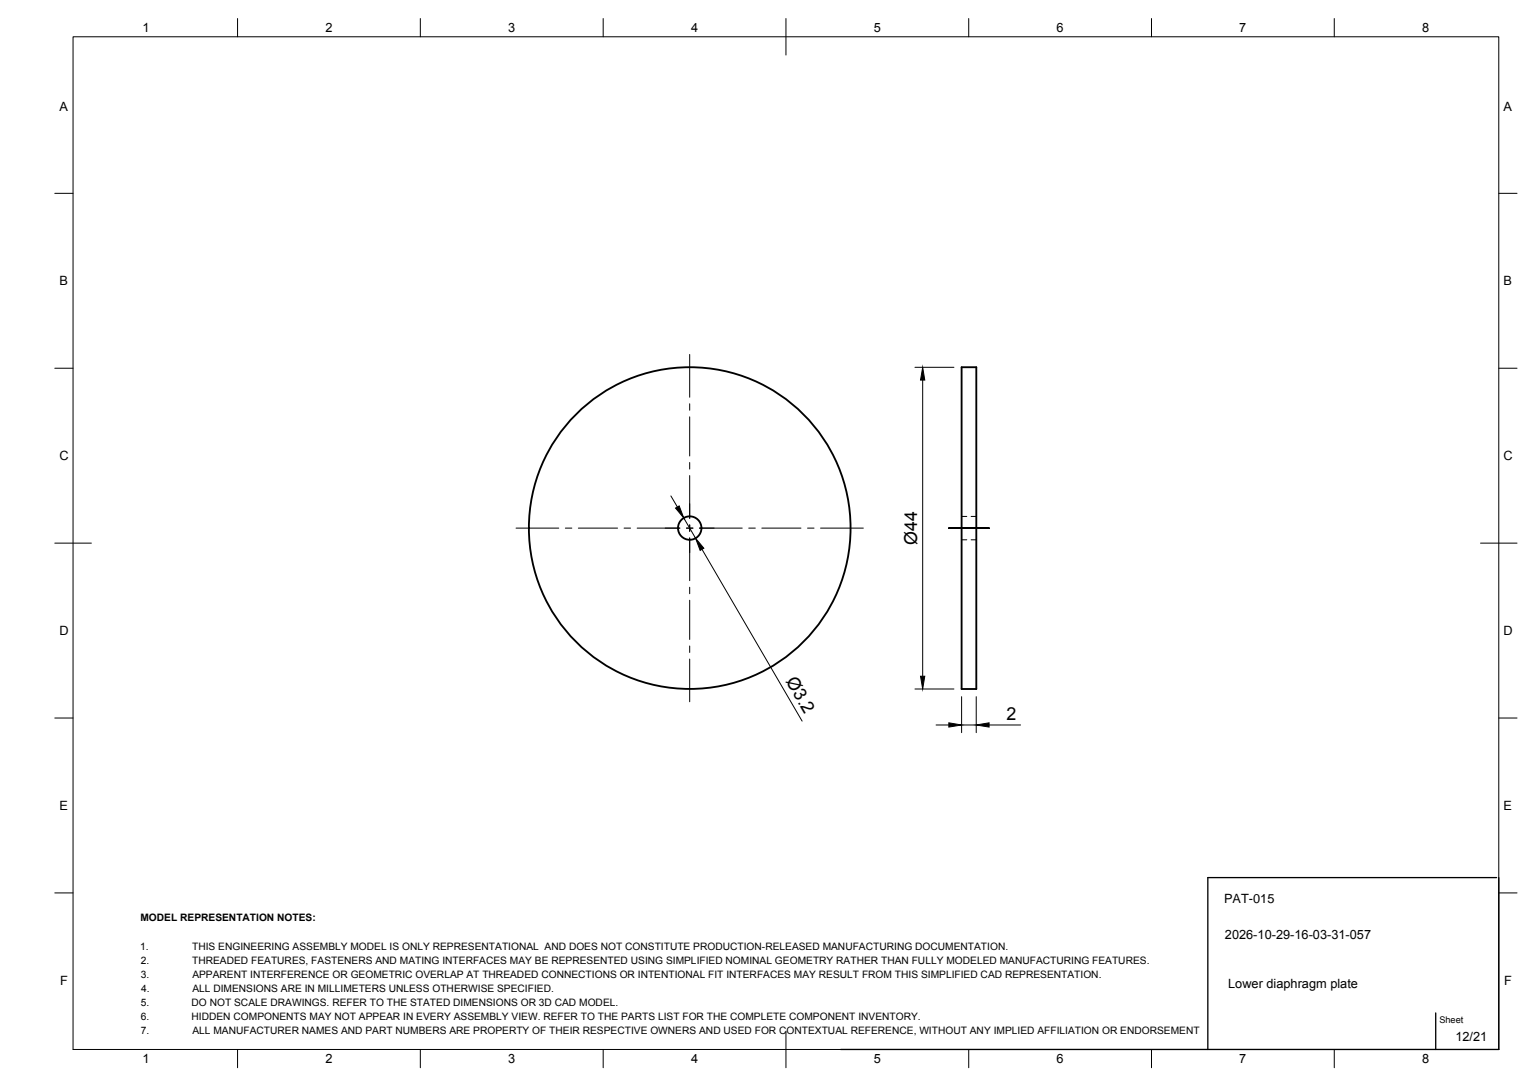
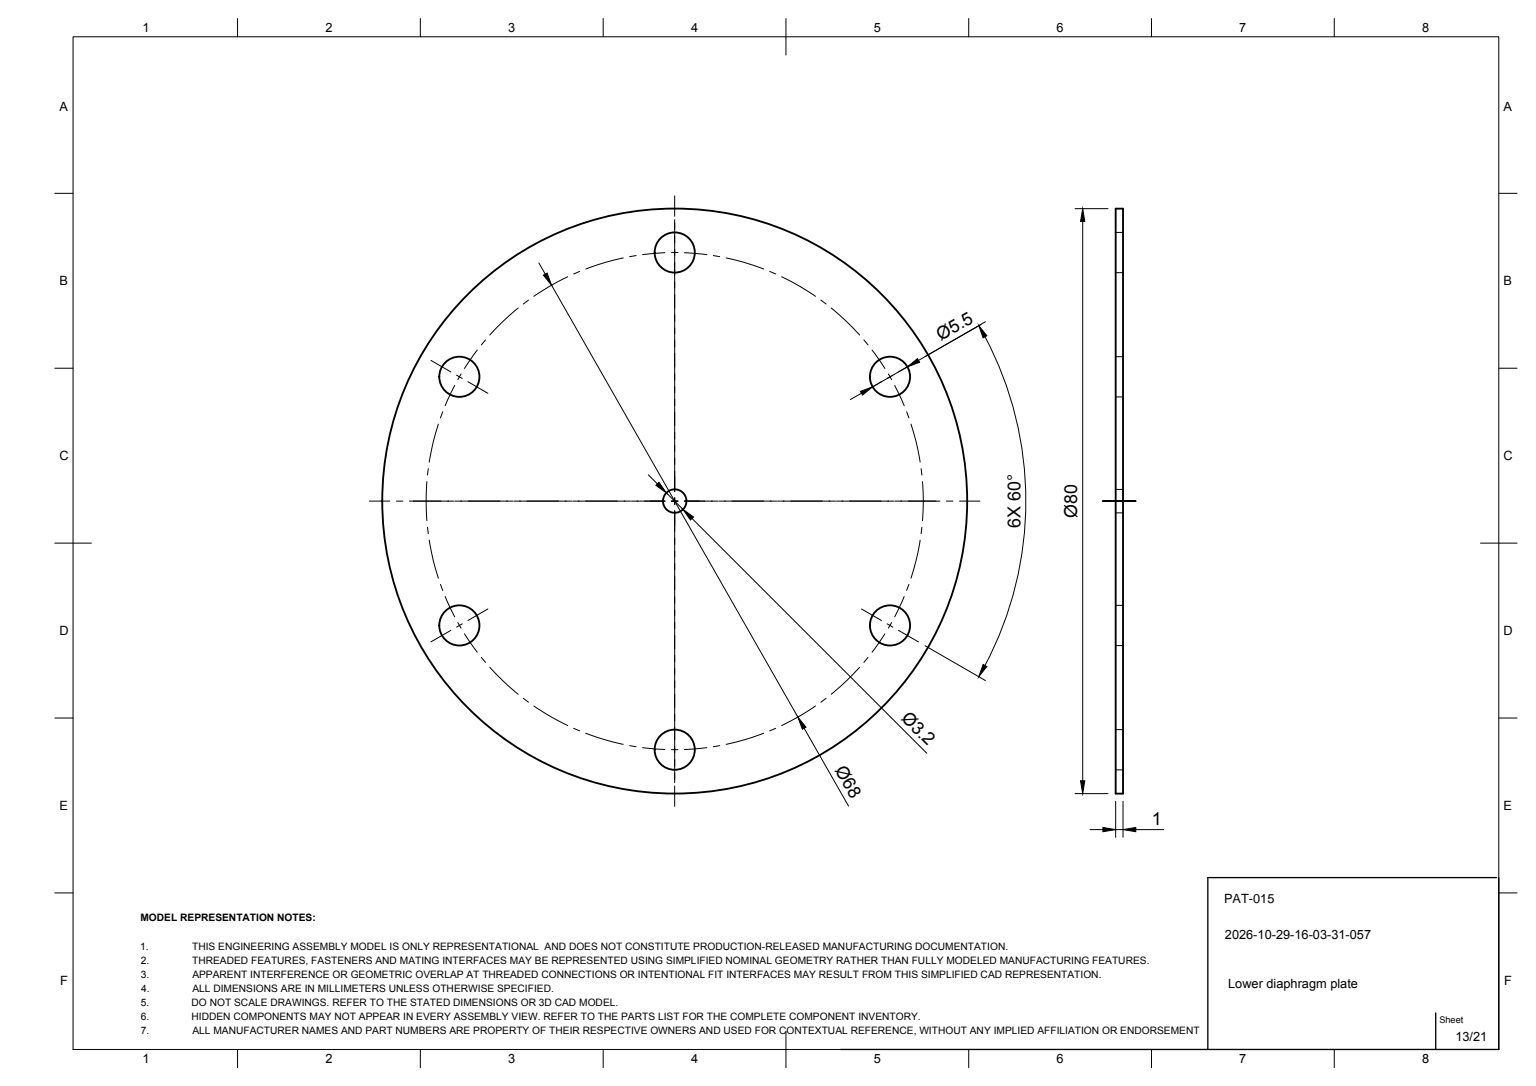
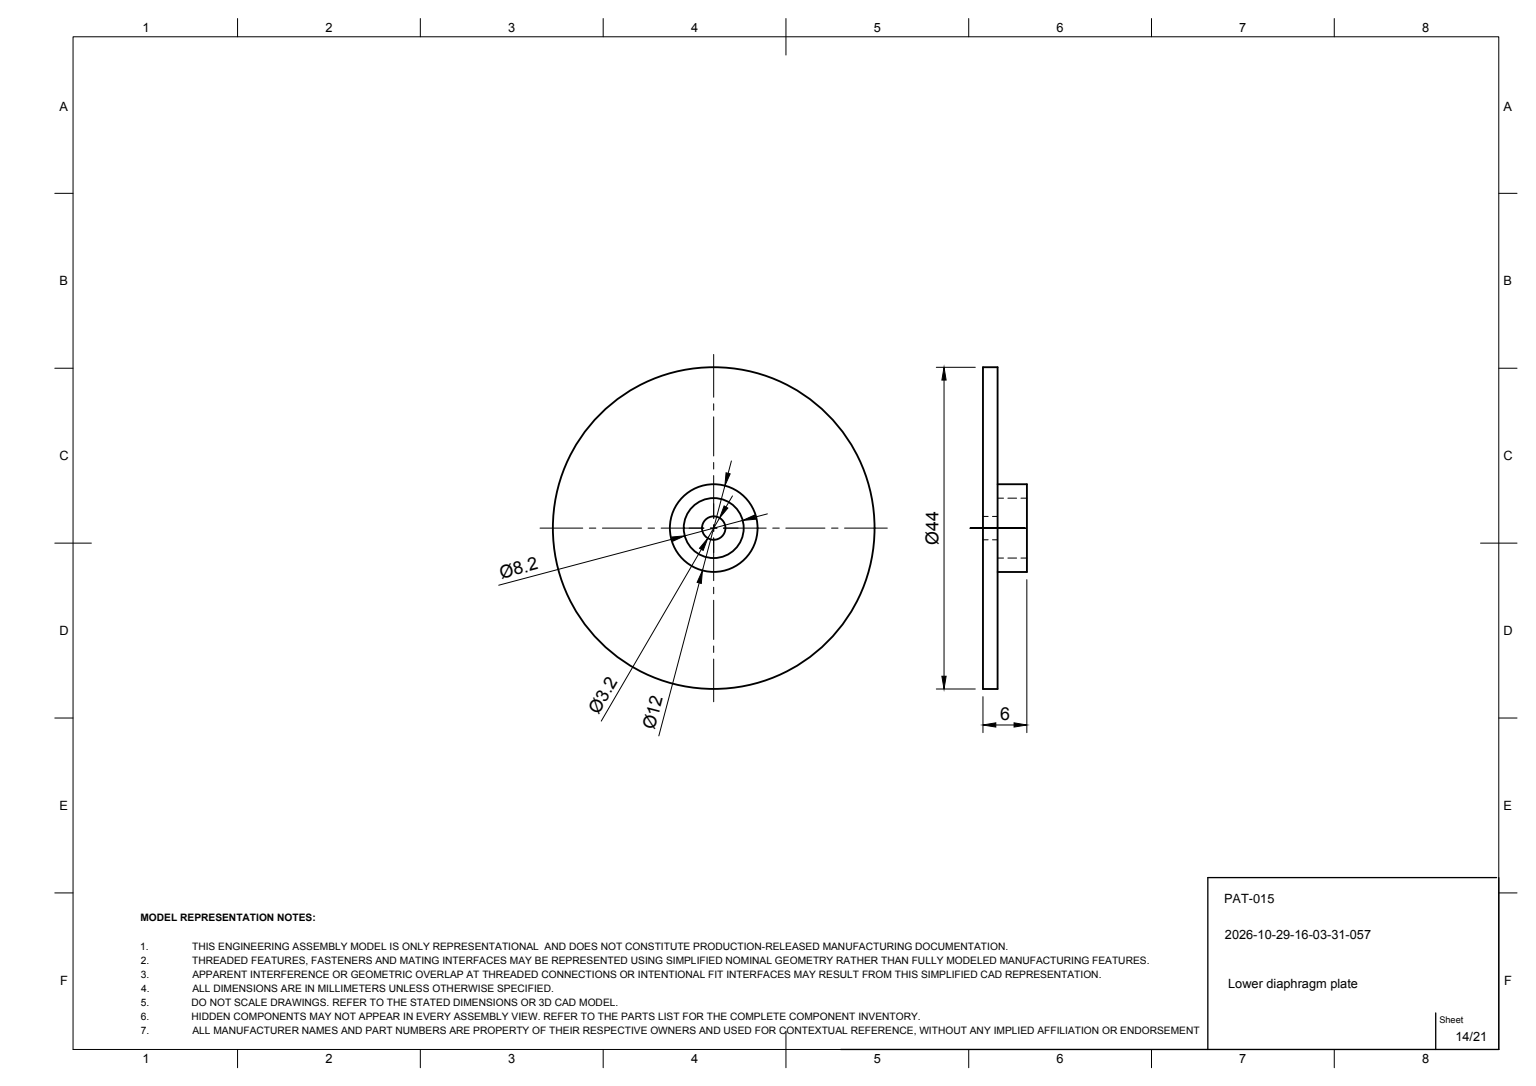
ISO-10303-21;
HEADER;
/* Generated by software containing ST-Developer
 * from STEP Tools, Inc. (www.steptools.com) 
 */

FILE_DESCRIPTION(
/* description */ ('PAT-015'),
/* implementation_level */ '2;1');

FILE_NAME(
/* name */ 'Lower diaphragm plate.step',
/* time_stamp */ '2026-10-29T16:03:43-07:00',
/* author */ (''),
/* organization */ (''),
/* preprocessor_version */ 'ST-DEVELOPER v20.2',
/* originating_system */ 'Autodesk Translation Framework v15.17.0.0',
/* authorisation */ '');

FILE_SCHEMA (('AUTOMOTIVE_DESIGN { 1 0 10303 214 3 1 1 }'));
ENDSEC;

DATA;
#10=MECHANICAL_DESIGN_GEOMETRIC_PRESENTATION_REPRESENTATION('',(#240),#10266);
#192=SHAPE_REPRESENTATION_RELATIONSHIP('SRR','None',#10363,#215);
#215=ADVANCED_BREP_SHAPE_REPRESENTATION('',(#265),#10251);
#240=STYLED_ITEM('',(#10561),#265);
#265=MANIFOLD_SOLID_BREP('Body1',#4699);
#370=FACE_BOUND('',#1083,.T.);
#371=FACE_BOUND('',#1085,.T.);
#495=PLANE('',#5260);
#496=PLANE('',#5261);
#719=FACE_OUTER_BOUND('',#1080,.T.);
#720=FACE_OUTER_BOUND('',#1081,.T.);
#721=FACE_OUTER_BOUND('',#1082,.T.);
#722=FACE_OUTER_BOUND('',#1084,.T.);
#1080=EDGE_LOOP('',(#3747,#3748,#3749,#3750));
#1081=EDGE_LOOP('',(#3751,#3752,#3753,#3754));
#1082=EDGE_LOOP('',(#3755));
#1083=EDGE_LOOP('',(#3756));
#1084=EDGE_LOOP('',(#3757));
#1085=EDGE_LOOP('',(#3758));
#1466=LINE('',#8734,#1746);
#1467=LINE('',#8740,#1747);
#1746=VECTOR('',#6271,0.16);
#1747=VECTOR('',#6278,2.2);
#1995=CIRCLE('',#5255,0.16);
#1996=CIRCLE('',#5256,0.16);
#1997=CIRCLE('',#5258,2.2);
#1998=CIRCLE('',#5259,2.2);
#2329=VERTEX_POINT('',#8731);
#2330=VERTEX_POINT('',#8733);
#2331=VERTEX_POINT('',#8737);
#2332=VERTEX_POINT('',#8739);
#2829=EDGE_CURVE('',#2329,#2329,#1995,.T.);
#2830=EDGE_CURVE('',#2329,#2330,#1466,.T.);
#2831=EDGE_CURVE('',#2330,#2330,#1996,.T.);
#2832=EDGE_CURVE('',#2331,#2331,#1997,.T.);
#2833=EDGE_CURVE('',#2331,#2332,#1467,.T.);
#2834=EDGE_CURVE('',#2332,#2332,#1998,.T.);
#3747=ORIENTED_EDGE('',*,*,#2829,.F.);
#3748=ORIENTED_EDGE('',*,*,#2830,.T.);
#3749=ORIENTED_EDGE('',*,*,#2831,.T.);
#3750=ORIENTED_EDGE('',*,*,#2830,.F.);
#3751=ORIENTED_EDGE('',*,*,#2832,.F.);
#3752=ORIENTED_EDGE('',*,*,#2833,.T.);
#3753=ORIENTED_EDGE('',*,*,#2834,.T.);
#3754=ORIENTED_EDGE('',*,*,#2833,.F.);
#3755=ORIENTED_EDGE('',*,*,#2832,.T.);
#3756=ORIENTED_EDGE('',*,*,#2829,.T.);
#3757=ORIENTED_EDGE('',*,*,#2834,.F.);
#3758=ORIENTED_EDGE('',*,*,#2831,.F.);
#4361=CYLINDRICAL_SURFACE('',#5254,0.16);
#4362=CYLINDRICAL_SURFACE('',#5257,2.2);
#4554=ADVANCED_FACE('',(#719),#4361,.F.);
#4555=ADVANCED_FACE('',(#720),#4362,.T.);
#4556=ADVANCED_FACE('',(#721,#370),#495,.T.);
#4557=ADVANCED_FACE('',(#722,#371),#496,.F.);
#4699=CLOSED_SHELL('',(#4554,#4555,#4556,#4557));
#5253=AXIS2_PLACEMENT_3D('',#8729,#6265,#6266);
#5254=AXIS2_PLACEMENT_3D('',#8730,#6267,#6268);
#5255=AXIS2_PLACEMENT_3D('',#8732,#6269,#6270);
#5256=AXIS2_PLACEMENT_3D('',#8735,#6272,#6273);
#5257=AXIS2_PLACEMENT_3D('',#8736,#6274,#6275);
#5258=AXIS2_PLACEMENT_3D('',#8738,#6276,#6277);
#5259=AXIS2_PLACEMENT_3D('',#8741,#6279,#6280);
#5260=AXIS2_PLACEMENT_3D('',#8742,#6281,#6282);
#5261=AXIS2_PLACEMENT_3D('',#8743,#6283,#6284);
#6265=DIRECTION('axis',(0.,0.,1.));
#6266=DIRECTION('refdir',(1.,0.,0.));
#6267=DIRECTION('center_axis',(0.,0.,1.));
#6268=DIRECTION('ref_axis',(1.,0.,0.));
#6269=DIRECTION('center_axis',(0.,0.,-1.));
#6270=DIRECTION('ref_axis',(1.,0.,0.));
#6271=DIRECTION('',(0.,0.,-1.));
#6272=DIRECTION('center_axis',(0.,0.,-1.));
#6273=DIRECTION('ref_axis',(1.,0.,0.));
#6274=DIRECTION('center_axis',(0.,0.,1.));
#6275=DIRECTION('ref_axis',(1.,0.,0.));
#6276=DIRECTION('center_axis',(0.,0.,1.));
#6277=DIRECTION('ref_axis',(1.,0.,0.));
#6278=DIRECTION('',(0.,0.,-1.));
#6279=DIRECTION('center_axis',(0.,0.,1.));
#6280=DIRECTION('ref_axis',(1.,0.,0.));
#6281=DIRECTION('center_axis',(0.,0.,1.));
#6282=DIRECTION('ref_axis',(1.,0.,0.));
#6283=DIRECTION('center_axis',(0.,0.,1.));
#6284=DIRECTION('ref_axis',(1.,0.,0.));
#8729=CARTESIAN_POINT('',(0.,0.,0.));
#8730=CARTESIAN_POINT('Origin',(0.,0.,4.8));
#8731=CARTESIAN_POINT('',(-0.16,-1.95943487863577E-17,5.));
#8732=CARTESIAN_POINT('Origin',(0.,0.,5.));
#8733=CARTESIAN_POINT('',(-0.16,-1.95943487863577E-17,4.8));
#8734=CARTESIAN_POINT('',(-0.16,-1.95943487863577E-17,4.8));
#8735=CARTESIAN_POINT('Origin',(0.,0.,4.8));
#8736=CARTESIAN_POINT('Origin',(0.,0.,4.8));
#8737=CARTESIAN_POINT('',(-2.2,-2.69422295812418E-16,5.));
#8738=CARTESIAN_POINT('Origin',(0.,0.,5.));
#8739=CARTESIAN_POINT('',(-2.2,-2.69422295812418E-16,4.8));
#8740=CARTESIAN_POINT('',(-2.2,-2.69422295812418E-16,4.8));
#8741=CARTESIAN_POINT('Origin',(0.,0.,4.8));
#8742=CARTESIAN_POINT('Origin',(0.,0.,5.));
#8743=CARTESIAN_POINT('Origin',(0.,0.,4.8));
#10226=UNCERTAINTY_MEASURE_WITH_UNIT(LENGTH_MEASURE(0.001),#10267,
'DISTANCE_ACCURACY_VALUE',
'Maximum model space distance between geometric entities at asserted c
onnectivities');
#10241=UNCERTAINTY_MEASURE_WITH_UNIT(LENGTH_MEASURE(0.001),#10267,
'DISTANCE_ACCURACY_VALUE',
'Maximum model space distance between geometric entities at asserted c
onnectivities');
#10251=(
GEOMETRIC_REPRESENTATION_CONTEXT(3)
GLOBAL_UNCERTAINTY_ASSIGNED_CONTEXT((#10226))
GLOBAL_UNIT_ASSIGNED_CONTEXT((#10267,#10269,#10270))
REPRESENTATION_CONTEXT('','3D')
);
#10266=(
GEOMETRIC_REPRESENTATION_CONTEXT(3)
GLOBAL_UNCERTAINTY_ASSIGNED_CONTEXT((#10241))
GLOBAL_UNIT_ASSIGNED_CONTEXT((#10267,#10269,#10270))
REPRESENTATION_CONTEXT('','3D')
);
#10267=(
LENGTH_UNIT()
NAMED_UNIT(*)
SI_UNIT(.CENTI.,.METRE.)
);
#10269=(
NAMED_UNIT(*)
PLANE_ANGLE_UNIT()
SI_UNIT($,.RADIAN.)
);
#10270=(
NAMED_UNIT(*)
SI_UNIT($,.STERADIAN.)
SOLID_ANGLE_UNIT()
);
#10280=SHAPE_DEFINITION_REPRESENTATION(#10304,#10363);
#10304=PRODUCT_DEFINITION_SHAPE('',$,#10388);
#10363=SHAPE_REPRESENTATION('',(#5253),#10251);
#10378=PRODUCT_DEFINITION_CONTEXT('part definition',#10452,'design');
#10388=PRODUCT_DEFINITION('Lower diaphragm plate',
'Lower diaphragm plate',#10412,#10378);
#10412=PRODUCT_DEFINITION_FORMATION('',$,#10463);
#10452=APPLICATION_CONTEXT(
'Core Data for Automotive Mechanical Design Process');
#10453=PRODUCT_CONTEXT('part definition',#10452,'mechanical');
#10463=PRODUCT('Lower diaphragm plate','Lower diaphragm plate',
'Lower diaphragm plate',(#10453));
#10555=COLOUR_RGB('Off White',0.89,0.88,0.83);
#10556=FILL_AREA_STYLE_COLOUR('',#10555);
#10557=FILL_AREA_STYLE('',(#10556));
#10558=SURFACE_STYLE_FILL_AREA(#10557);
#10559=SURFACE_SIDE_STYLE('',(#10558));
#10560=SURFACE_STYLE_USAGE(.BOTH.,#10559);
#10561=PRESENTATION_STYLE_ASSIGNMENT((#10560));
ENDSEC;
END-ISO-10303-21;
